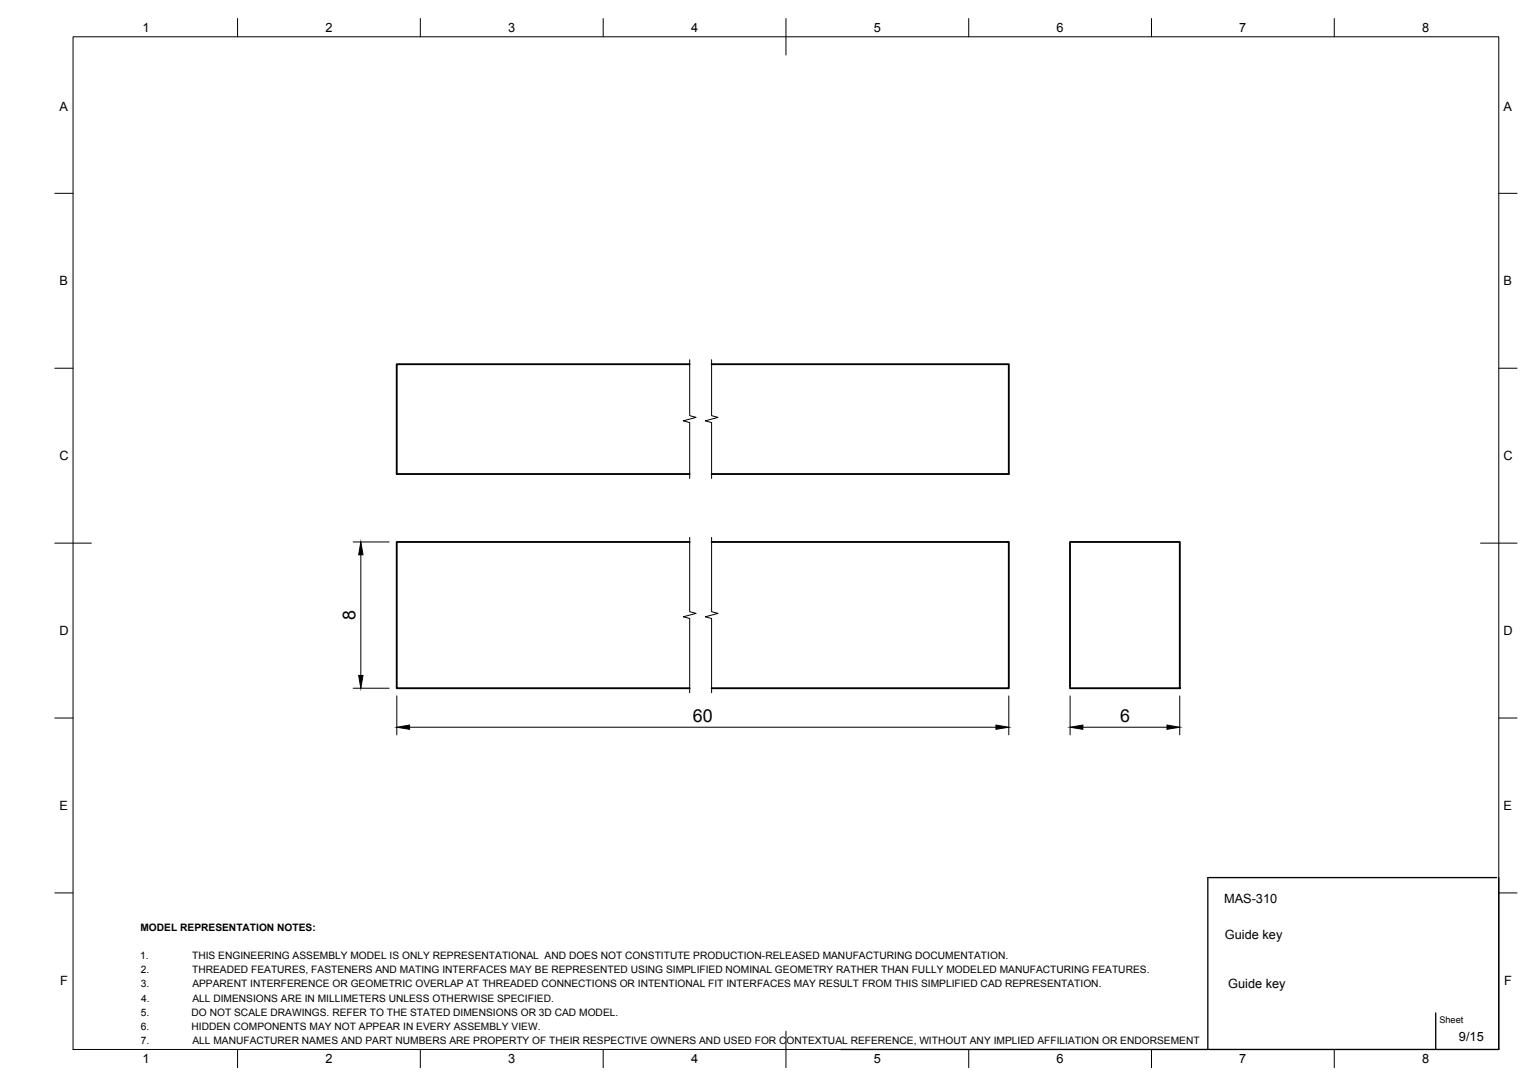
ISO-10303-21;
HEADER;
/* Generated by software containing ST-Developer
 * from STEP Tools, Inc. (www.steptools.com) 
 */

FILE_DESCRIPTION(
/* description */ ('Independent30mm screw-fed quill/spindle unit with16mm straight tool s
ocket, radial set screw, native reusable open ball bearings, retained 
inner/outer race stacks, keyed quill guide and M12x1.75 fine feed. Ext
ernal moving drive and tool not included. Ideal cage orbital links; in
dividual ball spin, force and preload not simulated. No drilling capac
ity, runout, speed, torque, load, life or machine safety rating.'),
/* implementation_level */ '2;1');

FILE_NAME(
/* name */ 'Guide key.step',
/* time_stamp */ '2026-11-08T18:59:42-08:00',
/* author */ (''),
/* organization */ (''),
/* preprocessor_version */ 'ST-DEVELOPER v20.2',
/* originating_system */ 'Autodesk Translation Framework v15.17.0.0',
/* authorisation */ '');

FILE_SCHEMA (('AUTOMOTIVE_DESIGN { 1 0 10303 214 3 1 1 }'));
ENDSEC;

DATA;
#10=MECHANICAL_DESIGN_GEOMETRIC_PRESENTATION_REPRESENTATION('',(#1598),#63898);
#1562=SHAPE_REPRESENTATION_RELATIONSHIP('SRR','None',#64001,#1580);
#1580=ADVANCED_BREP_SHAPE_REPRESENTATION('',(#1616),#63886);
#1598=STYLED_ITEM('',(#64098),#1616);
#1616=MANIFOLD_SOLID_BREP('Body1',#15484);
#3144=FACE_OUTER_BOUND('',#4027,.T.);
#3145=FACE_OUTER_BOUND('',#4028,.T.);
#3146=FACE_OUTER_BOUND('',#4029,.T.);
#3147=FACE_OUTER_BOUND('',#4030,.T.);
#3148=FACE_OUTER_BOUND('',#4031,.T.);
#3149=FACE_OUTER_BOUND('',#4032,.T.);
#4027=EDGE_LOOP('',(#12544,#12545,#12546,#12547));
#4028=EDGE_LOOP('',(#12548,#12549,#12550,#12551));
#4029=EDGE_LOOP('',(#12552,#12553,#12554,#12555));
#4030=EDGE_LOOP('',(#12556,#12557,#12558,#12559));
#4031=EDGE_LOOP('',(#12560,#12561,#12562,#12563));
#4032=EDGE_LOOP('',(#12564,#12565,#12566,#12567));
#4868=LINE('',#46816,#5631);
#4869=LINE('',#46818,#5632);
#4870=LINE('',#46820,#5633);
#4871=LINE('',#46821,#5634);
#4872=LINE('',#46824,#5635);
#4873=LINE('',#46826,#5636);
#4874=LINE('',#46827,#5637);
#4875=LINE('',#46830,#5638);
#4876=LINE('',#46832,#5639);
#4877=LINE('',#46833,#5640);
#4878=LINE('',#46835,#5641);
#4879=LINE('',#46836,#5642);
#5631=VECTOR('',#18512,10.);
#5632=VECTOR('',#18513,10.);
#5633=VECTOR('',#18514,10.);
#5634=VECTOR('',#18515,10.);
#5635=VECTOR('',#18518,10.);
#5636=VECTOR('',#18519,10.);
#5637=VECTOR('',#18520,10.);
#5638=VECTOR('',#18523,10.);
#5639=VECTOR('',#18524,10.);
#5640=VECTOR('',#18525,10.);
#5641=VECTOR('',#18528,10.);
#5642=VECTOR('',#18529,10.);
#6848=VERTEX_POINT('',#46814);
#6849=VERTEX_POINT('',#46815);
#6850=VERTEX_POINT('',#46817);
#6851=VERTEX_POINT('',#46819);
#6852=VERTEX_POINT('',#46823);
#6853=VERTEX_POINT('',#46825);
#6854=VERTEX_POINT('',#46829);
#6855=VERTEX_POINT('',#46831);
#8861=EDGE_CURVE('',#6848,#6849,#4868,.T.);
#8862=EDGE_CURVE('',#6849,#6850,#4869,.T.);
#8863=EDGE_CURVE('',#6851,#6850,#4870,.T.);
#8864=EDGE_CURVE('',#6848,#6851,#4871,.T.);
#8865=EDGE_CURVE('',#6852,#6848,#4872,.T.);
#8866=EDGE_CURVE('',#6853,#6851,#4873,.T.);
#8867=EDGE_CURVE('',#6852,#6853,#4874,.T.);
#8868=EDGE_CURVE('',#6854,#6852,#4875,.T.);
#8869=EDGE_CURVE('',#6855,#6853,#4876,.T.);
#8870=EDGE_CURVE('',#6854,#6855,#4877,.T.);
#8871=EDGE_CURVE('',#6849,#6854,#4878,.T.);
#8872=EDGE_CURVE('',#6850,#6855,#4879,.T.);
#12544=ORIENTED_EDGE('',*,*,#8861,.T.);
#12545=ORIENTED_EDGE('',*,*,#8862,.T.);
#12546=ORIENTED_EDGE('',*,*,#8863,.F.);
#12547=ORIENTED_EDGE('',*,*,#8864,.F.);
#12548=ORIENTED_EDGE('',*,*,#8865,.T.);
#12549=ORIENTED_EDGE('',*,*,#8864,.T.);
#12550=ORIENTED_EDGE('',*,*,#8866,.F.);
#12551=ORIENTED_EDGE('',*,*,#8867,.F.);
#12552=ORIENTED_EDGE('',*,*,#8868,.T.);
#12553=ORIENTED_EDGE('',*,*,#8867,.T.);
#12554=ORIENTED_EDGE('',*,*,#8869,.F.);
#12555=ORIENTED_EDGE('',*,*,#8870,.F.);
#12556=ORIENTED_EDGE('',*,*,#8871,.T.);
#12557=ORIENTED_EDGE('',*,*,#8870,.T.);
#12558=ORIENTED_EDGE('',*,*,#8872,.F.);
#12559=ORIENTED_EDGE('',*,*,#8862,.F.);
#12560=ORIENTED_EDGE('',*,*,#8872,.T.);
#12561=ORIENTED_EDGE('',*,*,#8869,.T.);
#12562=ORIENTED_EDGE('',*,*,#8866,.T.);
#12563=ORIENTED_EDGE('',*,*,#8863,.T.);
#12564=ORIENTED_EDGE('',*,*,#8871,.F.);
#12565=ORIENTED_EDGE('',*,*,#8861,.F.);
#12566=ORIENTED_EDGE('',*,*,#8865,.F.);
#12567=ORIENTED_EDGE('',*,*,#8868,.F.);
#14577=PLANE('',#16298);
#14578=PLANE('',#16299);
#14579=PLANE('',#16300);
#14580=PLANE('',#16301);
#14581=PLANE('',#16302);
#14582=PLANE('',#16303);
#15124=ADVANCED_FACE('',(#3144),#14577,.T.);
#15125=ADVANCED_FACE('',(#3145),#14578,.T.);
#15126=ADVANCED_FACE('',(#3146),#14579,.T.);
#15127=ADVANCED_FACE('',(#3147),#14580,.T.);
#15128=ADVANCED_FACE('',(#3148),#14581,.T.);
#15129=ADVANCED_FACE('',(#3149),#14582,.F.);
#15484=CLOSED_SHELL('',(#15124,#15125,#15126,#15127,#15128,#15129));
#16297=AXIS2_PLACEMENT_3D('',#46812,#18508,#18509);
#16298=AXIS2_PLACEMENT_3D('',#46813,#18510,#18511);
#16299=AXIS2_PLACEMENT_3D('',#46822,#18516,#18517);
#16300=AXIS2_PLACEMENT_3D('',#46828,#18521,#18522);
#16301=AXIS2_PLACEMENT_3D('',#46834,#18526,#18527);
#16302=AXIS2_PLACEMENT_3D('',#46837,#18530,#18531);
#16303=AXIS2_PLACEMENT_3D('',#46838,#18532,#18533);
#18508=DIRECTION('axis',(0.,0.,1.));
#18509=DIRECTION('refdir',(1.,0.,0.));
#18510=DIRECTION('center_axis',(0.,1.,0.));
#18511=DIRECTION('ref_axis',(-1.,0.,0.));
#18512=DIRECTION('',(-1.,0.,0.));
#18513=DIRECTION('',(0.,0.,1.));
#18514=DIRECTION('',(-1.,0.,0.));
#18515=DIRECTION('',(0.,0.,1.));
#18516=DIRECTION('center_axis',(1.,0.,0.));
#18517=DIRECTION('ref_axis',(0.,1.,0.));
#18518=DIRECTION('',(0.,1.,0.));
#18519=DIRECTION('',(0.,1.,0.));
#18520=DIRECTION('',(0.,0.,1.));
#18521=DIRECTION('center_axis',(0.,-1.,0.));
#18522=DIRECTION('ref_axis',(1.,0.,0.));
#18523=DIRECTION('',(1.,0.,0.));
#18524=DIRECTION('',(1.,0.,0.));
#18525=DIRECTION('',(0.,0.,1.));
#18526=DIRECTION('center_axis',(-1.,0.,0.));
#18527=DIRECTION('ref_axis',(0.,-1.,0.));
#18528=DIRECTION('',(0.,-1.,0.));
#18529=DIRECTION('',(0.,-1.,0.));
#18530=DIRECTION('center_axis',(0.,0.,1.));
#18531=DIRECTION('ref_axis',(1.,0.,0.));
#18532=DIRECTION('center_axis',(0.,0.,1.));
#18533=DIRECTION('ref_axis',(1.,0.,0.));
#46812=CARTESIAN_POINT('',(0.,0.,0.));
#46813=CARTESIAN_POINT('Origin',(-46.,3.,80.));
#46814=CARTESIAN_POINT('',(-46.,3.,80.));
#46815=CARTESIAN_POINT('',(-54.,3.,80.));
#46816=CARTESIAN_POINT('',(-46.,3.,80.));
#46817=CARTESIAN_POINT('',(-54.,3.,140.));
#46818=CARTESIAN_POINT('',(-54.,3.,80.));
#46819=CARTESIAN_POINT('',(-46.,3.,140.));
#46820=CARTESIAN_POINT('',(-46.,3.,140.));
#46821=CARTESIAN_POINT('',(-46.,3.,80.));
#46822=CARTESIAN_POINT('Origin',(-46.,-3.,80.));
#46823=CARTESIAN_POINT('',(-46.,-3.,80.));
#46824=CARTESIAN_POINT('',(-46.,-3.,80.));
#46825=CARTESIAN_POINT('',(-46.,-3.,140.));
#46826=CARTESIAN_POINT('',(-46.,-3.,140.));
#46827=CARTESIAN_POINT('',(-46.,-3.,80.));
#46828=CARTESIAN_POINT('Origin',(-54.,-3.,80.));
#46829=CARTESIAN_POINT('',(-54.,-3.,80.));
#46830=CARTESIAN_POINT('',(-54.,-3.,80.));
#46831=CARTESIAN_POINT('',(-54.,-3.,140.));
#46832=CARTESIAN_POINT('',(-54.,-3.,140.));
#46833=CARTESIAN_POINT('',(-54.,-3.,80.));
#46834=CARTESIAN_POINT('Origin',(-54.,3.,80.));
#46835=CARTESIAN_POINT('',(-54.,3.,80.));
#46836=CARTESIAN_POINT('',(-54.,3.,140.));
#46837=CARTESIAN_POINT('Origin',(-50.,0.,140.));
#46838=CARTESIAN_POINT('Origin',(-50.,0.,80.));
#63866=UNCERTAINTY_MEASURE_WITH_UNIT(LENGTH_MEASURE(0.01),#63899,
'DISTANCE_ACCURACY_VALUE',
'Maximum model space distance between geometric entities at asserted c
onnectivities');
#63878=UNCERTAINTY_MEASURE_WITH_UNIT(LENGTH_MEASURE(0.01),#63899,
'DISTANCE_ACCURACY_VALUE',
'Maximum model space distance between geometric entities at asserted c
onnectivities');
#63886=(
GEOMETRIC_REPRESENTATION_CONTEXT(3)
GLOBAL_UNCERTAINTY_ASSIGNED_CONTEXT((#63866))
GLOBAL_UNIT_ASSIGNED_CONTEXT((#63899,#63901,#63902))
REPRESENTATION_CONTEXT('','3D')
);
#63898=(
GEOMETRIC_REPRESENTATION_CONTEXT(3)
GLOBAL_UNCERTAINTY_ASSIGNED_CONTEXT((#63878))
GLOBAL_UNIT_ASSIGNED_CONTEXT((#63899,#63901,#63902))
REPRESENTATION_CONTEXT('','3D')
);
#63899=(
LENGTH_UNIT()
NAMED_UNIT(*)
SI_UNIT(.MILLI.,.METRE.)
);
#63901=(
NAMED_UNIT(*)
PLANE_ANGLE_UNIT()
SI_UNIT($,.RADIAN.)
);
#63902=(
NAMED_UNIT(*)
SI_UNIT($,.STERADIAN.)
SOLID_ANGLE_UNIT()
);
#63910=SHAPE_DEFINITION_REPRESENTATION(#63929,#64001);
#63929=PRODUCT_DEFINITION_SHAPE('',$,#64021);
#64001=SHAPE_REPRESENTATION('',(#16297),#63886);
#64013=PRODUCT_DEFINITION_CONTEXT('part definition',#64072,'design');
#64021=PRODUCT_DEFINITION('Guide key','Guide key',#64040,#64013);
#64040=PRODUCT_DEFINITION_FORMATION('',$,#64081);
#64072=APPLICATION_CONTEXT(
'Core Data for Automotive Mechanical Design Process');
#64073=PRODUCT_CONTEXT('part definition',#64072,'mechanical');
#64081=PRODUCT('Guide key','Guide key',$,(#64073));
#64098=PRESENTATION_STYLE_ASSIGNMENT((#64111));
#64111=SURFACE_STYLE_USAGE(.BOTH.,#64124);
#64124=SURFACE_SIDE_STYLE('',(#64137));
#64137=SURFACE_STYLE_FILL_AREA(#64150);
#64150=FILL_AREA_STYLE('Gray',(#64163));
#64163=FILL_AREA_STYLE_COLOUR('Gray',#64176);
#64176=COLOUR_RGB('Gray',0.407843137254902,0.447058823529412,0.498039215686275);
ENDSEC;
END-ISO-10303-21;
